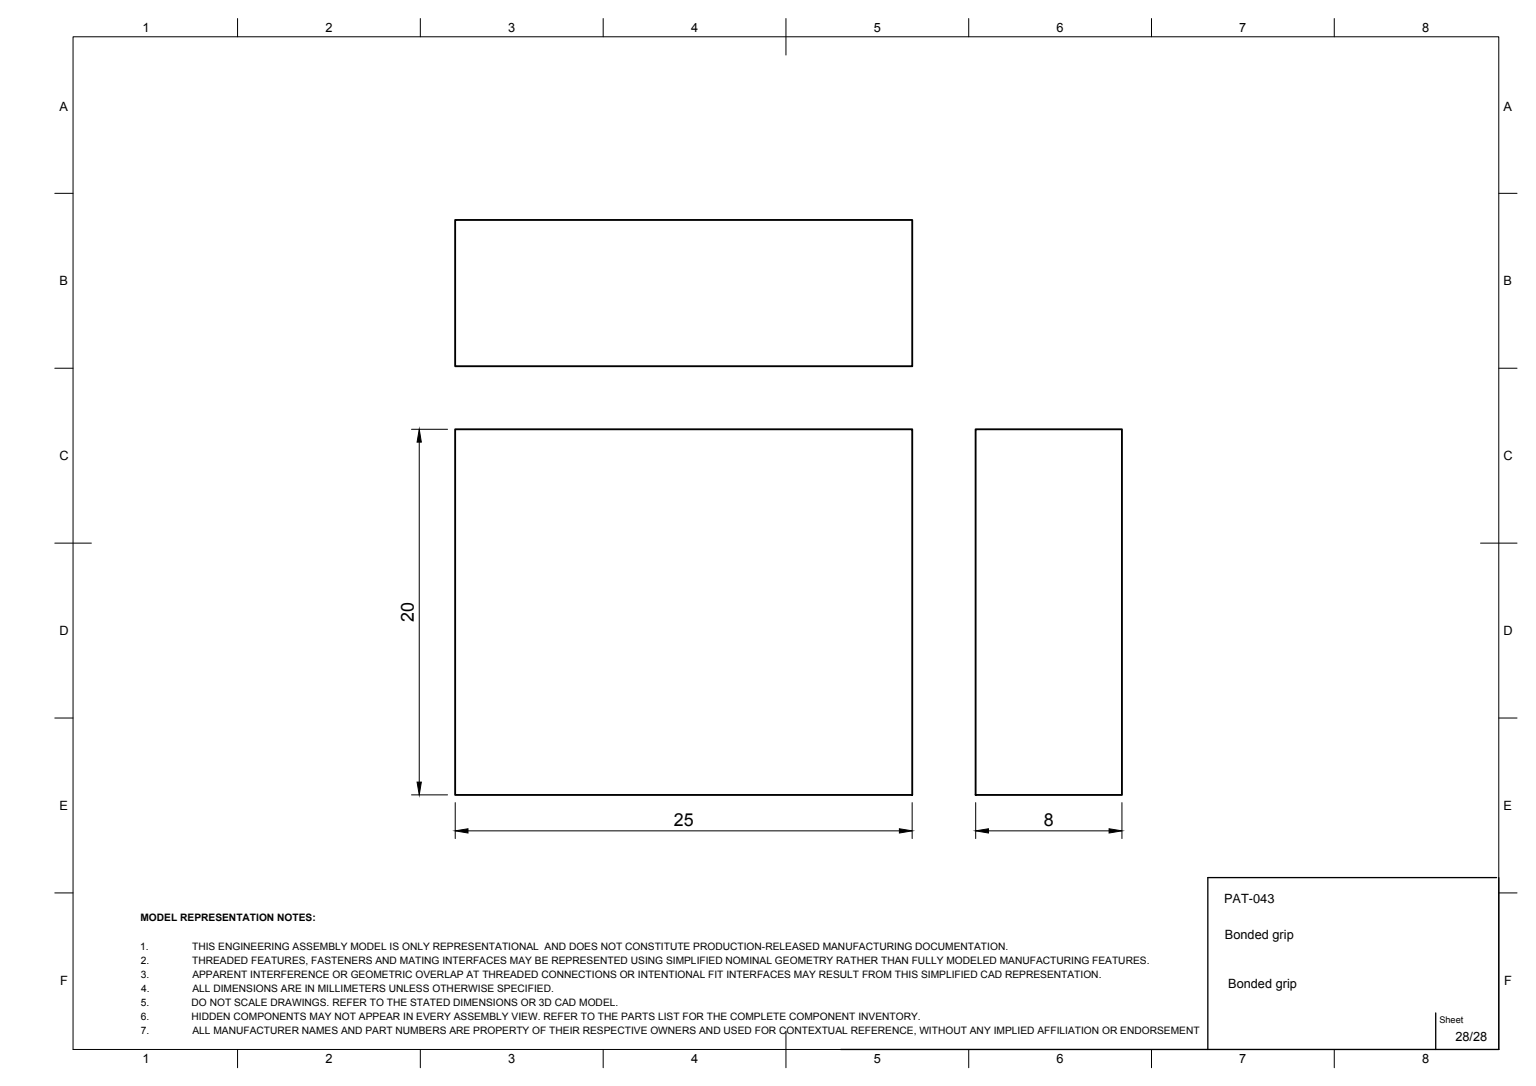
ISO-10303-21;
HEADER;
/* Generated by software containing ST-Developer
 * from STEP Tools, Inc. (www.steptools.com) 
 */

FILE_DESCRIPTION(
/* description */ ('Four-valve pipe header'),
/* implementation_level */ '2;1');

FILE_NAME(
/* name */ 'Bonded grip.step',
/* time_stamp */ '2026-10-29T16:56:19-07:00',
/* author */ (''),
/* organization */ (''),
/* preprocessor_version */ 'ST-DEVELOPER v20.2',
/* originating_system */ 'Autodesk Translation Framework v15.17.0.0',
/* authorisation */ '');

FILE_SCHEMA (('AUTOMOTIVE_DESIGN { 1 0 10303 214 3 1 1 }'));
ENDSEC;

DATA;
#10=MECHANICAL_DESIGN_GEOMETRIC_PRESENTATION_REPRESENTATION('',(#357),#10119);
#305=SHAPE_REPRESENTATION_RELATIONSHIP('SRR','None',#10268,#331);
#331=ADVANCED_BREP_SHAPE_REPRESENTATION('',(#381),#10117);
#357=STYLED_ITEM('',(#10477),#381);
#381=MANIFOLD_SOLID_BREP('Body1',#5605);
#730=PLANE('',#6483);
#731=PLANE('',#6484);
#732=PLANE('',#6485);
#733=PLANE('',#6486);
#734=PLANE('',#6487);
#735=PLANE('',#6488);
#1057=FACE_OUTER_BOUND('',#1497,.T.);
#1058=FACE_OUTER_BOUND('',#1498,.T.);
#1059=FACE_OUTER_BOUND('',#1499,.T.);
#1060=FACE_OUTER_BOUND('',#1500,.T.);
#1061=FACE_OUTER_BOUND('',#1501,.T.);
#1062=FACE_OUTER_BOUND('',#1502,.T.);
#1497=EDGE_LOOP('',(#5065,#5066,#5067,#5068));
#1498=EDGE_LOOP('',(#5069,#5070,#5071,#5072));
#1499=EDGE_LOOP('',(#5073,#5074,#5075,#5076));
#1500=EDGE_LOOP('',(#5077,#5078,#5079,#5080));
#1501=EDGE_LOOP('',(#5081,#5082,#5083,#5084));
#1502=EDGE_LOOP('',(#5085,#5086,#5087,#5088));
#1903=LINE('',#9913,#2321);
#1904=LINE('',#9915,#2322);
#1905=LINE('',#9917,#2323);
#1906=LINE('',#9918,#2324);
#1907=LINE('',#9921,#2325);
#1908=LINE('',#9923,#2326);
#1909=LINE('',#9924,#2327);
#1910=LINE('',#9927,#2328);
#1911=LINE('',#9929,#2329);
#1912=LINE('',#9930,#2330);
#1913=LINE('',#9932,#2331);
#1914=LINE('',#9933,#2332);
#2321=VECTOR('',#8130,1.);
#2322=VECTOR('',#8131,1.);
#2323=VECTOR('',#8132,1.);
#2324=VECTOR('',#8133,1.);
#2325=VECTOR('',#8136,1.);
#2326=VECTOR('',#8137,1.);
#2327=VECTOR('',#8138,1.);
#2328=VECTOR('',#8141,1.);
#2329=VECTOR('',#8142,1.);
#2330=VECTOR('',#8143,1.);
#2331=VECTOR('',#8146,1.);
#2332=VECTOR('',#8147,1.);
#3010=VERTEX_POINT('',#9911);
#3011=VERTEX_POINT('',#9912);
#3012=VERTEX_POINT('',#9914);
#3013=VERTEX_POINT('',#9916);
#3014=VERTEX_POINT('',#9920);
#3015=VERTEX_POINT('',#9922);
#3016=VERTEX_POINT('',#9926);
#3017=VERTEX_POINT('',#9928);
#3699=EDGE_CURVE('',#3010,#3011,#1903,.T.);
#3700=EDGE_CURVE('',#3011,#3012,#1904,.T.);
#3701=EDGE_CURVE('',#3013,#3012,#1905,.T.);
#3702=EDGE_CURVE('',#3010,#3013,#1906,.T.);
#3703=EDGE_CURVE('',#3014,#3010,#1907,.T.);
#3704=EDGE_CURVE('',#3015,#3013,#1908,.T.);
#3705=EDGE_CURVE('',#3014,#3015,#1909,.T.);
#3706=EDGE_CURVE('',#3016,#3014,#1910,.T.);
#3707=EDGE_CURVE('',#3017,#3015,#1911,.T.);
#3708=EDGE_CURVE('',#3016,#3017,#1912,.T.);
#3709=EDGE_CURVE('',#3011,#3016,#1913,.T.);
#3710=EDGE_CURVE('',#3012,#3017,#1914,.T.);
#5065=ORIENTED_EDGE('',*,*,#3699,.T.);
#5066=ORIENTED_EDGE('',*,*,#3700,.T.);
#5067=ORIENTED_EDGE('',*,*,#3701,.F.);
#5068=ORIENTED_EDGE('',*,*,#3702,.F.);
#5069=ORIENTED_EDGE('',*,*,#3703,.T.);
#5070=ORIENTED_EDGE('',*,*,#3702,.T.);
#5071=ORIENTED_EDGE('',*,*,#3704,.F.);
#5072=ORIENTED_EDGE('',*,*,#3705,.F.);
#5073=ORIENTED_EDGE('',*,*,#3706,.T.);
#5074=ORIENTED_EDGE('',*,*,#3705,.T.);
#5075=ORIENTED_EDGE('',*,*,#3707,.F.);
#5076=ORIENTED_EDGE('',*,*,#3708,.F.);
#5077=ORIENTED_EDGE('',*,*,#3709,.T.);
#5078=ORIENTED_EDGE('',*,*,#3708,.T.);
#5079=ORIENTED_EDGE('',*,*,#3710,.F.);
#5080=ORIENTED_EDGE('',*,*,#3700,.F.);
#5081=ORIENTED_EDGE('',*,*,#3710,.T.);
#5082=ORIENTED_EDGE('',*,*,#3707,.T.);
#5083=ORIENTED_EDGE('',*,*,#3704,.T.);
#5084=ORIENTED_EDGE('',*,*,#3701,.T.);
#5085=ORIENTED_EDGE('',*,*,#3709,.F.);
#5086=ORIENTED_EDGE('',*,*,#3699,.F.);
#5087=ORIENTED_EDGE('',*,*,#3703,.F.);
#5088=ORIENTED_EDGE('',*,*,#3706,.F.);
#5557=ADVANCED_FACE('',(#1057),#730,.T.);
#5558=ADVANCED_FACE('',(#1058),#731,.T.);
#5559=ADVANCED_FACE('',(#1059),#732,.T.);
#5560=ADVANCED_FACE('',(#1060),#733,.T.);
#5561=ADVANCED_FACE('',(#1061),#734,.T.);
#5562=ADVANCED_FACE('',(#1062),#735,.F.);
#5605=CLOSED_SHELL('',(#5557,#5558,#5559,#5560,#5561,#5562));
#6482=AXIS2_PLACEMENT_3D('',#9909,#8126,#8127);
#6483=AXIS2_PLACEMENT_3D('',#9910,#8128,#8129);
#6484=AXIS2_PLACEMENT_3D('',#9919,#8134,#8135);
#6485=AXIS2_PLACEMENT_3D('',#9925,#8139,#8140);
#6486=AXIS2_PLACEMENT_3D('',#9931,#8144,#8145);
#6487=AXIS2_PLACEMENT_3D('',#9934,#8148,#8149);
#6488=AXIS2_PLACEMENT_3D('',#9935,#8150,#8151);
#8126=DIRECTION('axis',(0.,0.,1.));
#8127=DIRECTION('refdir',(1.,0.,0.));
#8128=DIRECTION('center_axis',(0.,1.,0.));
#8129=DIRECTION('ref_axis',(-1.,0.,0.));
#8130=DIRECTION('',(-1.,0.,0.));
#8131=DIRECTION('',(0.,0.,1.));
#8132=DIRECTION('',(-1.,0.,0.));
#8133=DIRECTION('',(0.,0.,1.));
#8134=DIRECTION('center_axis',(1.,0.,0.));
#8135=DIRECTION('ref_axis',(0.,1.,0.));
#8136=DIRECTION('',(0.,1.,0.));
#8137=DIRECTION('',(0.,1.,0.));
#8138=DIRECTION('',(0.,0.,1.));
#8139=DIRECTION('center_axis',(0.,-1.,0.));
#8140=DIRECTION('ref_axis',(1.,0.,0.));
#8141=DIRECTION('',(1.,0.,0.));
#8142=DIRECTION('',(1.,0.,0.));
#8143=DIRECTION('',(0.,0.,1.));
#8144=DIRECTION('center_axis',(-1.,0.,0.));
#8145=DIRECTION('ref_axis',(0.,-1.,0.));
#8146=DIRECTION('',(0.,-1.,0.));
#8147=DIRECTION('',(0.,-1.,0.));
#8148=DIRECTION('center_axis',(0.,0.,1.));
#8149=DIRECTION('ref_axis',(1.,0.,0.));
#8150=DIRECTION('center_axis',(0.,0.,1.));
#8151=DIRECTION('ref_axis',(1.,0.,0.));
#9909=CARTESIAN_POINT('',(0.,0.,0.));
#9910=CARTESIAN_POINT('Origin',(8.5,1.,9.4));
#9911=CARTESIAN_POINT('',(8.5,1.,9.4));
#9912=CARTESIAN_POINT('',(6.,1.,9.4));
#9913=CARTESIAN_POINT('',(8.5,1.,9.4));
#9914=CARTESIAN_POINT('',(6.,1.,10.2));
#9915=CARTESIAN_POINT('',(6.,1.,9.4));
#9916=CARTESIAN_POINT('',(8.5,1.,10.2));
#9917=CARTESIAN_POINT('',(8.5,1.,10.2));
#9918=CARTESIAN_POINT('',(8.5,1.,9.4));
#9919=CARTESIAN_POINT('Origin',(8.5,-1.,9.4));
#9920=CARTESIAN_POINT('',(8.5,-1.,9.4));
#9921=CARTESIAN_POINT('',(8.5,-1.,9.4));
#9922=CARTESIAN_POINT('',(8.5,-1.,10.2));
#9923=CARTESIAN_POINT('',(8.5,-1.,10.2));
#9924=CARTESIAN_POINT('',(8.5,-1.,9.4));
#9925=CARTESIAN_POINT('Origin',(6.,-1.,9.4));
#9926=CARTESIAN_POINT('',(6.,-1.,9.4));
#9927=CARTESIAN_POINT('',(6.,-1.,9.4));
#9928=CARTESIAN_POINT('',(6.,-1.,10.2));
#9929=CARTESIAN_POINT('',(6.,-1.,10.2));
#9930=CARTESIAN_POINT('',(6.,-1.,9.4));
#9931=CARTESIAN_POINT('Origin',(6.,1.,9.4));
#9932=CARTESIAN_POINT('',(6.,1.,9.4));
#9933=CARTESIAN_POINT('',(6.,1.,10.2));
#9934=CARTESIAN_POINT('Origin',(7.25,0.,10.2));
#9935=CARTESIAN_POINT('Origin',(7.25,0.,9.4));
#10086=UNCERTAINTY_MEASURE_WITH_UNIT(LENGTH_MEASURE(0.001),#10120,
'DISTANCE_ACCURACY_VALUE',
'Maximum model space distance between geometric entities at asserted c
onnectivities');
#10088=UNCERTAINTY_MEASURE_WITH_UNIT(LENGTH_MEASURE(0.001),#10120,
'DISTANCE_ACCURACY_VALUE',
'Maximum model space distance between geometric entities at asserted c
onnectivities');
#10117=(
GEOMETRIC_REPRESENTATION_CONTEXT(3)
GLOBAL_UNCERTAINTY_ASSIGNED_CONTEXT((#10086))
GLOBAL_UNIT_ASSIGNED_CONTEXT((#10120,#10122,#10123))
REPRESENTATION_CONTEXT('','3D')
);
#10119=(
GEOMETRIC_REPRESENTATION_CONTEXT(3)
GLOBAL_UNCERTAINTY_ASSIGNED_CONTEXT((#10088))
GLOBAL_UNIT_ASSIGNED_CONTEXT((#10120,#10122,#10123))
REPRESENTATION_CONTEXT('','3D')
);
#10120=(
LENGTH_UNIT()
NAMED_UNIT(*)
SI_UNIT(.CENTI.,.METRE.)
);
#10122=(
NAMED_UNIT(*)
PLANE_ANGLE_UNIT()
SI_UNIT($,.RADIAN.)
);
#10123=(
NAMED_UNIT(*)
SI_UNIT($,.STERADIAN.)
SOLID_ANGLE_UNIT()
);
#10152=SHAPE_DEFINITION_REPRESENTATION(#10182,#10268);
#10182=PRODUCT_DEFINITION_SHAPE('',$,#10299);
#10268=SHAPE_REPRESENTATION('',(#6482),#10117);
#10270=PRODUCT_DEFINITION_CONTEXT('part definition',#10362,'design');
#10299=PRODUCT_DEFINITION('Bonded grip','Bonded grip',#10329,#10270);
#10329=PRODUCT_DEFINITION_FORMATION('',$,#10392);
#10362=APPLICATION_CONTEXT(
'Core Data for Automotive Mechanical Design Process');
#10363=PRODUCT_CONTEXT('part definition',#10362,'mechanical');
#10392=PRODUCT('Bonded grip','Bonded grip','Bonded grip',(#10363));
#10471=COLOUR_RGB('Black',0.12,0.14,0.17);
#10472=FILL_AREA_STYLE_COLOUR('',#10471);
#10473=FILL_AREA_STYLE('',(#10472));
#10474=SURFACE_STYLE_FILL_AREA(#10473);
#10475=SURFACE_SIDE_STYLE('',(#10474));
#10476=SURFACE_STYLE_USAGE(.BOTH.,#10475);
#10477=PRESENTATION_STYLE_ASSIGNMENT((#10476));
ENDSEC;
END-ISO-10303-21;
